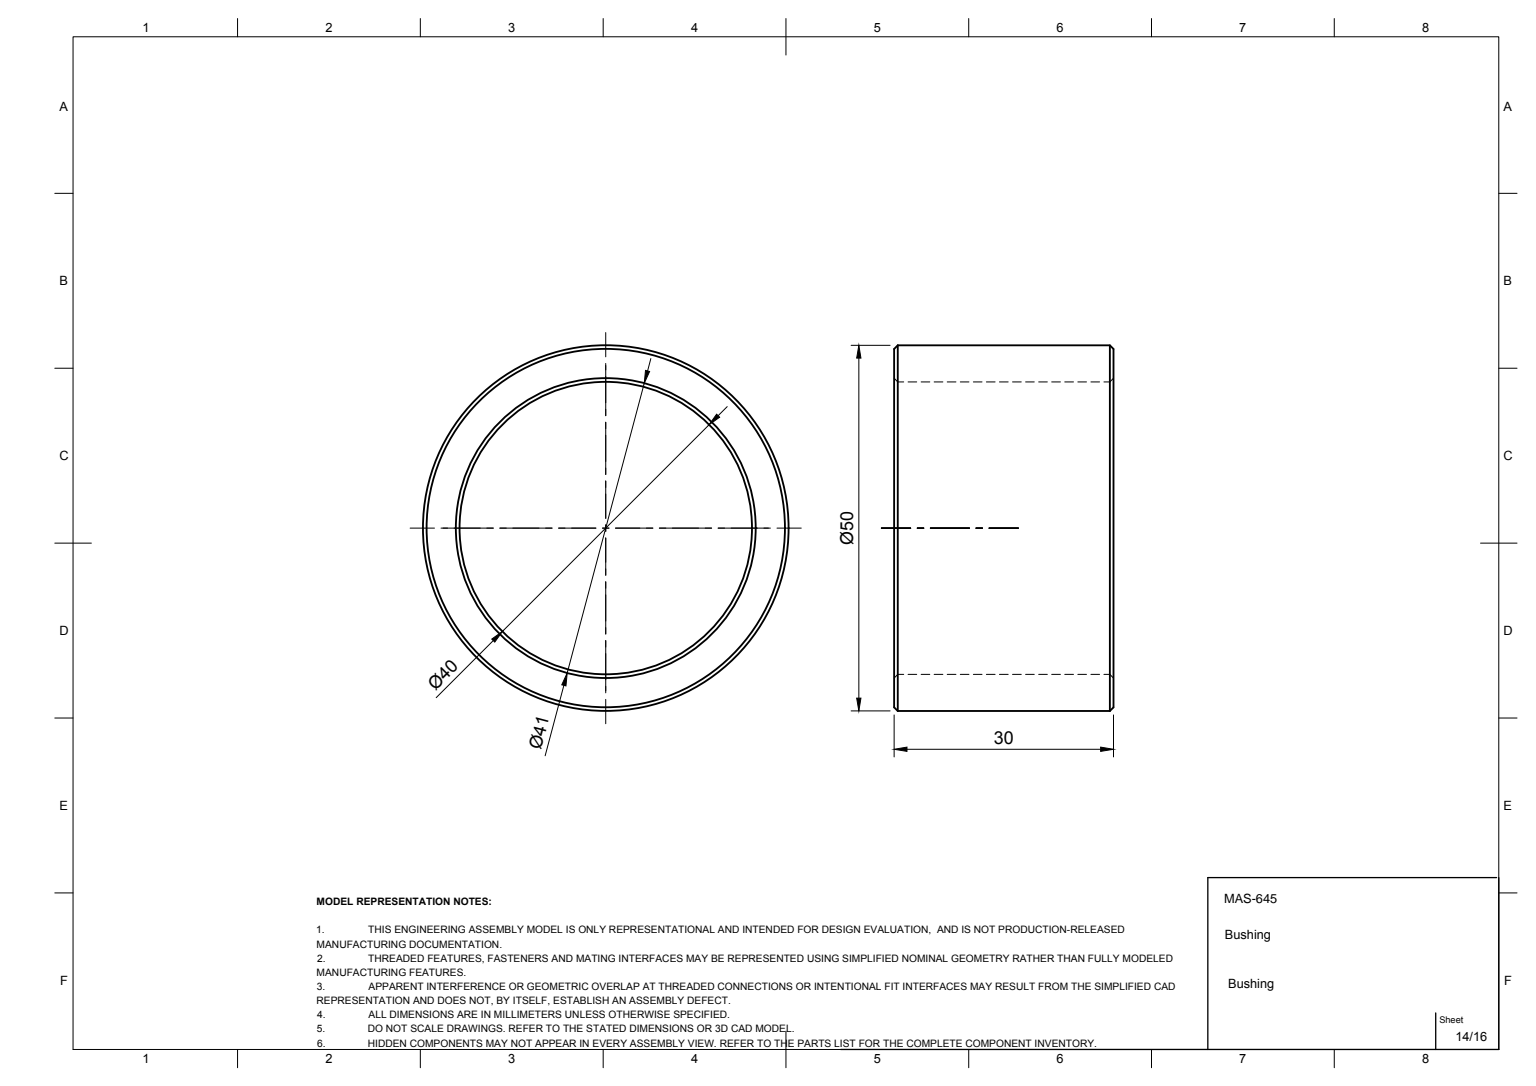
ISO-10303-21;
HEADER;
FILE_DESCRIPTION((''),'2;1');
FILE_NAME('Bushing.step','2026-10-09T10:54:55-07:00',(''),(''),'','','');
FILE_SCHEMA (('AUTOMOTIVE_DESIGN { 1 0 10303 214 3 1 1 }'));
ENDSEC;
DATA;
#10=MECHANICAL_DESIGN_GEOMETRIC_PRESENTATION_REPRESENTATION('',(#604),#63824);
#574=SHAPE_REPRESENTATION_RELATIONSHIP('SRR','None',#63888,#589) ;
#589=ADVANCED_BREP_SHAPE_REPRESENTATION('',(#619),#63818) ;
#604=STYLED_ITEM('',(#63963),#619) ;
#619=MANIFOLD_SOLID_BREP('Body1',#15503) ;
#755=FACE_BOUND('',#3205,.T.) ;
#756=FACE_BOUND('',#3210,.T.) ;
#1036=PLANE('',#17214) ;
#1037=PLANE('',#17223) ;
#1508=CYLINDRICAL_SURFACE('',#17208,20.) ;
#1509=CYLINDRICAL_SURFACE('',#17219,25.) ;
#2211=FACE_OUTER_BOUND('',#3202,.T.) ;
#2212=FACE_OUTER_BOUND('',#3203,.T.) ;
#2213=FACE_OUTER_BOUND('',#3204,.T.) ;
#2214=FACE_OUTER_BOUND('',#3206,.T.) ;
#2215=FACE_OUTER_BOUND('',#3207,.T.) ;
#2216=FACE_OUTER_BOUND('',#3208,.T.) ;
#2217=FACE_OUTER_BOUND('',#3209,.T.) ;
#2218=FACE_OUTER_BOUND('',#3211,.T.) ;
#3202=EDGE_LOOP('',(#12816,#12817,#12818,#12819,#12820)) ;
#3203=EDGE_LOOP('',(#12821,#12822,#12823,#12824)) ;
#3204=EDGE_LOOP('',(#12825)) ;
#3205=EDGE_LOOP('',(#12826)) ;
#3206=EDGE_LOOP('',(#12827,#12828,#12829,#12830,#12831)) ;
#3207=EDGE_LOOP('',(#12832,#12833,#12834,#12835,#12836)) ;
#3208=EDGE_LOOP('',(#12837,#12838,#12839,#12840)) ;
#3209=EDGE_LOOP('',(#12841)) ;
#3210=EDGE_LOOP('',(#12842)) ;
#3211=EDGE_LOOP('',(#12843,#12844,#12845,#12846,#12847)) ;
#4329=CIRCLE('',#17209,20.) ;
#4330=CIRCLE('',#17210,20.) ;
#4331=CIRCLE('',#17211,20.) ;
#4332=CIRCLE('',#17213,20.5) ;
#4333=CIRCLE('',#17215,24.5) ;
#4334=CIRCLE('',#17217,25.) ;
#4335=CIRCLE('',#17218,25.) ;
#4336=CIRCLE('',#17220,25.) ;
#4337=CIRCLE('',#17222,24.5) ;
#4338=CIRCLE('',#17224,20.5) ;
#5223=LINE('',#53720,#5879) ;
#5224=LINE('',#53724,#5880) ;
#5225=LINE('',#53733,#5881) ;
#5226=LINE('',#53737,#5882) ;
#5227=LINE('',#53741,#5883) ;
#5228=LINE('',#53747,#5884) ;
#5879=VECTOR('',#21507,20.) ;
#5880=VECTOR('',#21512,20.) ;
#5881=VECTOR('',#21523,24.5) ;
#5882=VECTOR('',#21528,25.) ;
#5883=VECTOR('',#21533,25.) ;
#5884=VECTOR('',#21542,20.5) ;
#6941=VERTEX_POINT('',#53715) ;
#6942=VERTEX_POINT('',#53716) ;
#6943=VERTEX_POINT('',#53719) ;
#6944=VERTEX_POINT('',#53723) ;
#6945=VERTEX_POINT('',#53727) ;
#6946=VERTEX_POINT('',#53730) ;
#6947=VERTEX_POINT('',#53731) ;
#6948=VERTEX_POINT('',#53736) ;
#6949=VERTEX_POINT('',#53740) ;
#6950=VERTEX_POINT('',#53744) ;
#8962=EDGE_CURVE('',#6941,#6942,#4329,.T.) ;
#8963=EDGE_CURVE('',#6942,#6941,#4330,.T.) ;
#8964=EDGE_CURVE('',#6942,#6943,#5223,.T.) ;
#8965=EDGE_CURVE('',#6943,#6943,#4331,.T.) ;
#8966=EDGE_CURVE('',#6943,#6944,#5224,.T.) ;
#8967=EDGE_CURVE('',#6944,#6944,#4332,.T.) ;
#8968=EDGE_CURVE('',#6945,#6945,#4333,.T.) ;
#8969=EDGE_CURVE('',#6946,#6947,#4334,.T.) ;
#8970=EDGE_CURVE('',#6947,#6945,#5225,.T.) ;
#8971=EDGE_CURVE('',#6947,#6946,#4335,.T.) ;
#8972=EDGE_CURVE('',#6946,#6948,#5226,.T.) ;
#8973=EDGE_CURVE('',#6948,#6948,#4336,.T.) ;
#8974=EDGE_CURVE('',#6948,#6949,#5227,.T.) ;
#8975=EDGE_CURVE('',#6949,#6949,#4337,.T.) ;
#8976=EDGE_CURVE('',#6950,#6950,#4338,.T.) ;
#8977=EDGE_CURVE('',#6941,#6950,#5228,.T.) ;
#12816=ORIENTED_EDGE('',*,*,#8962,.F.) ;
#12817=ORIENTED_EDGE('',*,*,#8963,.F.) ;
#12818=ORIENTED_EDGE('',*,*,#8964,.T.) ;
#12819=ORIENTED_EDGE('',*,*,#8965,.T.) ;
#12820=ORIENTED_EDGE('',*,*,#8964,.F.) ;
#12821=ORIENTED_EDGE('',*,*,#8965,.F.) ;
#12822=ORIENTED_EDGE('',*,*,#8966,.T.) ;
#12823=ORIENTED_EDGE('',*,*,#8967,.T.) ;
#12824=ORIENTED_EDGE('',*,*,#8966,.F.) ;
#12825=ORIENTED_EDGE('',*,*,#8968,.T.) ;
#12826=ORIENTED_EDGE('',*,*,#8967,.F.) ;
#12827=ORIENTED_EDGE('',*,*,#8969,.T.) ;
#12828=ORIENTED_EDGE('',*,*,#8970,.T.) ;
#12829=ORIENTED_EDGE('',*,*,#8968,.F.) ;
#12830=ORIENTED_EDGE('',*,*,#8970,.F.) ;
#12831=ORIENTED_EDGE('',*,*,#8971,.T.) ;
#12832=ORIENTED_EDGE('',*,*,#8969,.F.) ;
#12833=ORIENTED_EDGE('',*,*,#8972,.T.) ;
#12834=ORIENTED_EDGE('',*,*,#8973,.T.) ;
#12835=ORIENTED_EDGE('',*,*,#8972,.F.) ;
#12836=ORIENTED_EDGE('',*,*,#8971,.F.) ;
#12837=ORIENTED_EDGE('',*,*,#8973,.F.) ;
#12838=ORIENTED_EDGE('',*,*,#8974,.T.) ;
#12839=ORIENTED_EDGE('',*,*,#8975,.T.) ;
#12840=ORIENTED_EDGE('',*,*,#8974,.F.) ;
#12841=ORIENTED_EDGE('',*,*,#8975,.F.) ;
#12842=ORIENTED_EDGE('',*,*,#8976,.T.) ;
#12843=ORIENTED_EDGE('',*,*,#8962,.T.) ;
#12844=ORIENTED_EDGE('',*,*,#8963,.T.) ;
#12845=ORIENTED_EDGE('',*,*,#8977,.T.) ;
#12846=ORIENTED_EDGE('',*,*,#8976,.F.) ;
#12847=ORIENTED_EDGE('',*,*,#8977,.F.) ;
#14559=CONICAL_SURFACE('',#17212,20.,0.785398163397449) ;
#14560=CONICAL_SURFACE('',#17216,24.5,0.785398163397449) ;
#14561=CONICAL_SURFACE('',#17221,25.,0.785398163397448) ;
#14562=CONICAL_SURFACE('',#17225,20.5,0.785398163397448) ;
#15299=ADVANCED_FACE('',(#2211),#1508,.F.) ;
#15300=ADVANCED_FACE('',(#2212),#14559,.F.) ;
#15301=ADVANCED_FACE('',(#2213,#755),#1036,.T.) ;
#15302=ADVANCED_FACE('',(#2214),#14560,.T.) ;
#15303=ADVANCED_FACE('',(#2215),#1509,.T.) ;
#15304=ADVANCED_FACE('',(#2216),#14561,.T.) ;
#15305=ADVANCED_FACE('',(#2217,#756),#1037,.T.) ;
#15306=ADVANCED_FACE('',(#2218),#14562,.F.) ;
#15503=CLOSED_SHELL('',(#15299,#15300,#15301,#15302,#15303,#15304,#15305,
#15306)) ;
#17207=AXIS2_PLACEMENT_3D('',#53713,#21499,#21500) ;
#17208=AXIS2_PLACEMENT_3D('',#53714,#21501,#21502) ;
#17209=AXIS2_PLACEMENT_3D('',#53717,#21503,#21504) ;
#17210=AXIS2_PLACEMENT_3D('',#53718,#21505,#21506) ;
#17211=AXIS2_PLACEMENT_3D('',#53721,#21508,#21509) ;
#17212=AXIS2_PLACEMENT_3D('',#53722,#21510,#21511) ;
#17213=AXIS2_PLACEMENT_3D('',#53725,#21513,#21514) ;
#17214=AXIS2_PLACEMENT_3D('',#53726,#21515,#21516) ;
#17215=AXIS2_PLACEMENT_3D('',#53728,#21517,#21518) ;
#17216=AXIS2_PLACEMENT_3D('',#53729,#21519,#21520) ;
#17217=AXIS2_PLACEMENT_3D('',#53732,#21521,#21522) ;
#17218=AXIS2_PLACEMENT_3D('',#53734,#21524,#21525) ;
#17219=AXIS2_PLACEMENT_3D('',#53735,#21526,#21527) ;
#17220=AXIS2_PLACEMENT_3D('',#53738,#21529,#21530) ;
#17221=AXIS2_PLACEMENT_3D('',#53739,#21531,#21532) ;
#17222=AXIS2_PLACEMENT_3D('',#53742,#21534,#21535) ;
#17223=AXIS2_PLACEMENT_3D('',#53743,#21536,#21537) ;
#17224=AXIS2_PLACEMENT_3D('',#53745,#21538,#21539) ;
#17225=AXIS2_PLACEMENT_3D('',#53746,#21540,#21541) ;
#21499=DIRECTION('axis',(0.,0.,1.)) ;
#21500=DIRECTION('refdir',(1.,0.,0.)) ;
#21501=DIRECTION('center_axis',(-1.,-6.12323399573677E-17,0.)) ;
#21502=DIRECTION('ref_axis',(6.12323399573677E-17,-1.,0.)) ;
#21503=DIRECTION('center_axis',(-1.,-6.12323399573677E-17,0.)) ;
#21504=DIRECTION('ref_axis',(6.12323399573677E-17,-1.,0.)) ;
#21505=DIRECTION('center_axis',(-1.,-6.12323399573677E-17,0.)) ;
#21506=DIRECTION('ref_axis',(6.12323399573677E-17,-1.,0.)) ;
#21507=DIRECTION('',(-1.,-6.12323399573677E-17,0.)) ;
#21508=DIRECTION('center_axis',(-1.,-6.12323399573677E-17,0.)) ;
#21509=DIRECTION('ref_axis',(6.12323399573677E-17,-1.,0.)) ;
#21510=DIRECTION('center_axis',(-1.,-6.12323399573677E-17,0.)) ;
#21511=DIRECTION('ref_axis',(6.12323399573677E-17,-1.,0.)) ;
#21512=DIRECTION('',(-0.707106781186547,0.707106781186548,-8.65956056235494E-17)) ;
#21513=DIRECTION('center_axis',(-1.,-6.12323399573677E-17,0.)) ;
#21514=DIRECTION('ref_axis',(6.12323399573677E-17,-1.,0.)) ;
#21515=DIRECTION('center_axis',(-1.,-6.12323399573677E-17,0.)) ;
#21516=DIRECTION('ref_axis',(6.12323399573677E-17,-1.,0.)) ;
#21517=DIRECTION('center_axis',(-1.,-6.12323399573677E-17,0.)) ;
#21518=DIRECTION('ref_axis',(6.12323399573677E-17,-1.,0.)) ;
#21519=DIRECTION('center_axis',(1.,6.12323399573677E-17,0.)) ;
#21520=DIRECTION('ref_axis',(-6.12323399573677E-17,1.,0.)) ;
#21521=DIRECTION('center_axis',(-1.,-6.12323399573677E-17,0.)) ;
#21522=DIRECTION('ref_axis',(6.12323399573677E-17,-1.,0.)) ;
#21523=DIRECTION('',(-0.707106781186547,0.707106781186548,8.65956056235494E-17)) ;
#21524=DIRECTION('center_axis',(-1.,-6.12323399573677E-17,0.)) ;
#21525=DIRECTION('ref_axis',(6.12323399573677E-17,-1.,0.)) ;
#21526=DIRECTION('center_axis',(-1.,-6.12323399573677E-17,0.)) ;
#21527=DIRECTION('ref_axis',(6.12323399573677E-17,-1.,0.)) ;
#21528=DIRECTION('',(1.,6.12323399573677E-17,0.)) ;
#21529=DIRECTION('center_axis',(-1.,-6.12323399573677E-17,0.)) ;
#21530=DIRECTION('ref_axis',(6.12323399573677E-17,-1.,0.)) ;
#21531=DIRECTION('center_axis',(-1.,-6.12323399573677E-17,0.)) ;
#21532=DIRECTION('ref_axis',(6.12323399573677E-17,-1.,0.)) ;
#21533=DIRECTION('',(0.707106781186548,-0.707106781186547,8.65956056235493E-17)) ;
#21534=DIRECTION('center_axis',(-1.,-6.12323399573677E-17,0.)) ;
#21535=DIRECTION('ref_axis',(6.12323399573677E-17,-1.,0.)) ;
#21536=DIRECTION('center_axis',(1.,6.12323399573677E-17,0.)) ;
#21537=DIRECTION('ref_axis',(-6.12323399573677E-17,1.,0.)) ;
#21538=DIRECTION('center_axis',(-1.,-6.12323399573677E-17,0.)) ;
#21539=DIRECTION('ref_axis',(6.12323399573677E-17,-1.,0.)) ;
#21540=DIRECTION('center_axis',(1.,6.12323399573677E-17,0.)) ;
#21541=DIRECTION('ref_axis',(-6.12323399573677E-17,1.,0.)) ;
#21542=DIRECTION('',(0.707106781186548,-0.707106781186547,-8.65956056235493E-17)) ;
#53713=CARTESIAN_POINT('',(0.,0.,0.)) ;
#53714=CARTESIAN_POINT('Origin',(-3.,-1.83697019872103E-16,0.)) ;
#53715=CARTESIAN_POINT('',(29.5,-20.,0.)) ;
#53716=CARTESIAN_POINT('',(29.5,20.,-2.44929359829471E-15)) ;
#53717=CARTESIAN_POINT('Origin',(29.5,1.80635402874235E-15,0.)) ;
#53718=CARTESIAN_POINT('Origin',(29.5,1.80635402874235E-15,0.)) ;
#53719=CARTESIAN_POINT('',(0.499999999999999,20.,-2.44929359829471E-15)) ;
#53720=CARTESIAN_POINT('',(-3.,20.,-2.44929359829471E-15)) ;
#53721=CARTESIAN_POINT('Origin',(0.5,3.06161699786838E-17,0.)) ;
#53722=CARTESIAN_POINT('Origin',(0.5,3.06161699786838E-17,0.)) ;
#53723=CARTESIAN_POINT('',(-2.28983498828939E-15,20.5,-2.51052593825207E-15)) ;
#53724=CARTESIAN_POINT('',(0.499999999999999,20.,-2.44929359829471E-15)) ;
#53725=CARTESIAN_POINT('Origin',(0.,0.,0.)) ;
#53726=CARTESIAN_POINT('Origin',(1.27815278805432E-15,-20.5,0.)) ;
#53727=CARTESIAN_POINT('',(1.50019232895551E-15,-24.5,0.)) ;
#53728=CARTESIAN_POINT('Origin',(0.,0.,0.)) ;
#53729=CARTESIAN_POINT('Origin',(0.,0.,0.)) ;
#53730=CARTESIAN_POINT('',(0.499999999999998,25.,-3.06161699786838E-15)) ;
#53731=CARTESIAN_POINT('',(0.500000000000001,-25.,-3.06161699786838E-15)) ;
#53732=CARTESIAN_POINT('Origin',(0.5,3.06161699786838E-17,0.)) ;
#53733=CARTESIAN_POINT('',(1.50019232895551E-15,-24.5,-3.00038465791102E-15)) ;
#53734=CARTESIAN_POINT('Origin',(0.5,3.06161699786838E-17,0.)) ;
#53735=CARTESIAN_POINT('Origin',(-3.,-1.83697019872103E-16,0.)) ;
#53736=CARTESIAN_POINT('',(29.5,25.,-3.06161699786838E-15)) ;
#53737=CARTESIAN_POINT('',(-3.,25.,-3.06161699786838E-15)) ;
#53738=CARTESIAN_POINT('Origin',(29.5,1.80635402874235E-15,0.)) ;
#53739=CARTESIAN_POINT('Origin',(29.5,1.80635402874235E-15,0.)) ;
#53740=CARTESIAN_POINT('',(30.,24.5,-3.00038465791102E-15)) ;
#53741=CARTESIAN_POINT('',(29.5,25.,-3.06161699786838E-15)) ;
#53742=CARTESIAN_POINT('Origin',(30.,1.83697019872103E-15,0.)) ;
#53743=CARTESIAN_POINT('Origin',(30.,-24.5,0.)) ;
#53744=CARTESIAN_POINT('',(30.,-20.5,0.)) ;
#53745=CARTESIAN_POINT('Origin',(30.,1.83697019872103E-15,0.)) ;
#53746=CARTESIAN_POINT('Origin',(30.,1.83697019872103E-15,0.)) ;
#53747=CARTESIAN_POINT('',(30.,-20.5,-2.51052593825207E-15)) ;
#63801=UNCERTAINTY_MEASURE_WITH_UNIT(LENGTH_MEASURE(0.01),#63825,
'DISTANCE_ACCURACY_VALUE',
'Maximum model space distance between geometric entities at asserted c
onnectivities') ;
#63807=UNCERTAINTY_MEASURE_WITH_UNIT(LENGTH_MEASURE(0.01),#63825,
'DISTANCE_ACCURACY_VALUE',
'Maximum model space distance between geometric entities at asserted c
onnectivities') ;
#63818=(
GEOMETRIC_REPRESENTATION_CONTEXT(3)
GLOBAL_UNCERTAINTY_ASSIGNED_CONTEXT((#63801))
GLOBAL_UNIT_ASSIGNED_CONTEXT((#63825,#63827,#63828))
REPRESENTATION_CONTEXT('','3D')
) ;
#63824=(
GEOMETRIC_REPRESENTATION_CONTEXT(3)
GLOBAL_UNCERTAINTY_ASSIGNED_CONTEXT((#63807))
GLOBAL_UNIT_ASSIGNED_CONTEXT((#63825,#63827,#63828))
REPRESENTATION_CONTEXT('','3D')
) ;
#63825=(
LENGTH_UNIT()
NAMED_UNIT(*)
SI_UNIT(.MILLI.,.METRE.)
) ;
#63827=(
NAMED_UNIT(*)
PLANE_ANGLE_UNIT()
SI_UNIT($,.RADIAN.)
) ;
#63828=(
NAMED_UNIT(*)
SI_UNIT($,.STERADIAN.)
SOLID_ANGLE_UNIT()
) ;
#63839=SHAPE_DEFINITION_REPRESENTATION(#63855,#63888) ;
#63855=PRODUCT_DEFINITION_SHAPE('',$,#63905) ;
#63888=SHAPE_REPRESENTATION('',(#17207),#63818) ;
#63894=PRODUCT_DEFINITION_CONTEXT('part definition',#63944,'design') ;
#63905=PRODUCT_DEFINITION('Bushing','Bushing',#63921,#63894) ;
#63921=PRODUCT_DEFINITION_FORMATION('',$,#63956) ;
#63944=APPLICATION_CONTEXT(
'Core Data for Automotive Mechanical Design Process') ;
#63945=PRODUCT_CONTEXT('part definition',#63944,'mechanical') ;
#63956=PRODUCT('Bushing','Bushing',$,(#63945)) ;
#63963=PRESENTATION_STYLE_ASSIGNMENT((#63968)) ;
#63968=SURFACE_STYLE_USAGE(.BOTH.,#63973) ;
#63973=SURFACE_SIDE_STYLE('',(#63978)) ;
#63978=SURFACE_STYLE_FILL_AREA(#63983) ;
#63983=FILL_AREA_STYLE('Opaque(160,160,160)',(#63988)) ;
#63988=FILL_AREA_STYLE_COLOUR('Opaque(160,160,160)',#63993) ;
#63993=COLOUR_RGB('Opaque(160,160,160)', 0.09019608, 0.27058824, 0.51372549) ;
ENDSEC;
END-ISO-10303-21;
